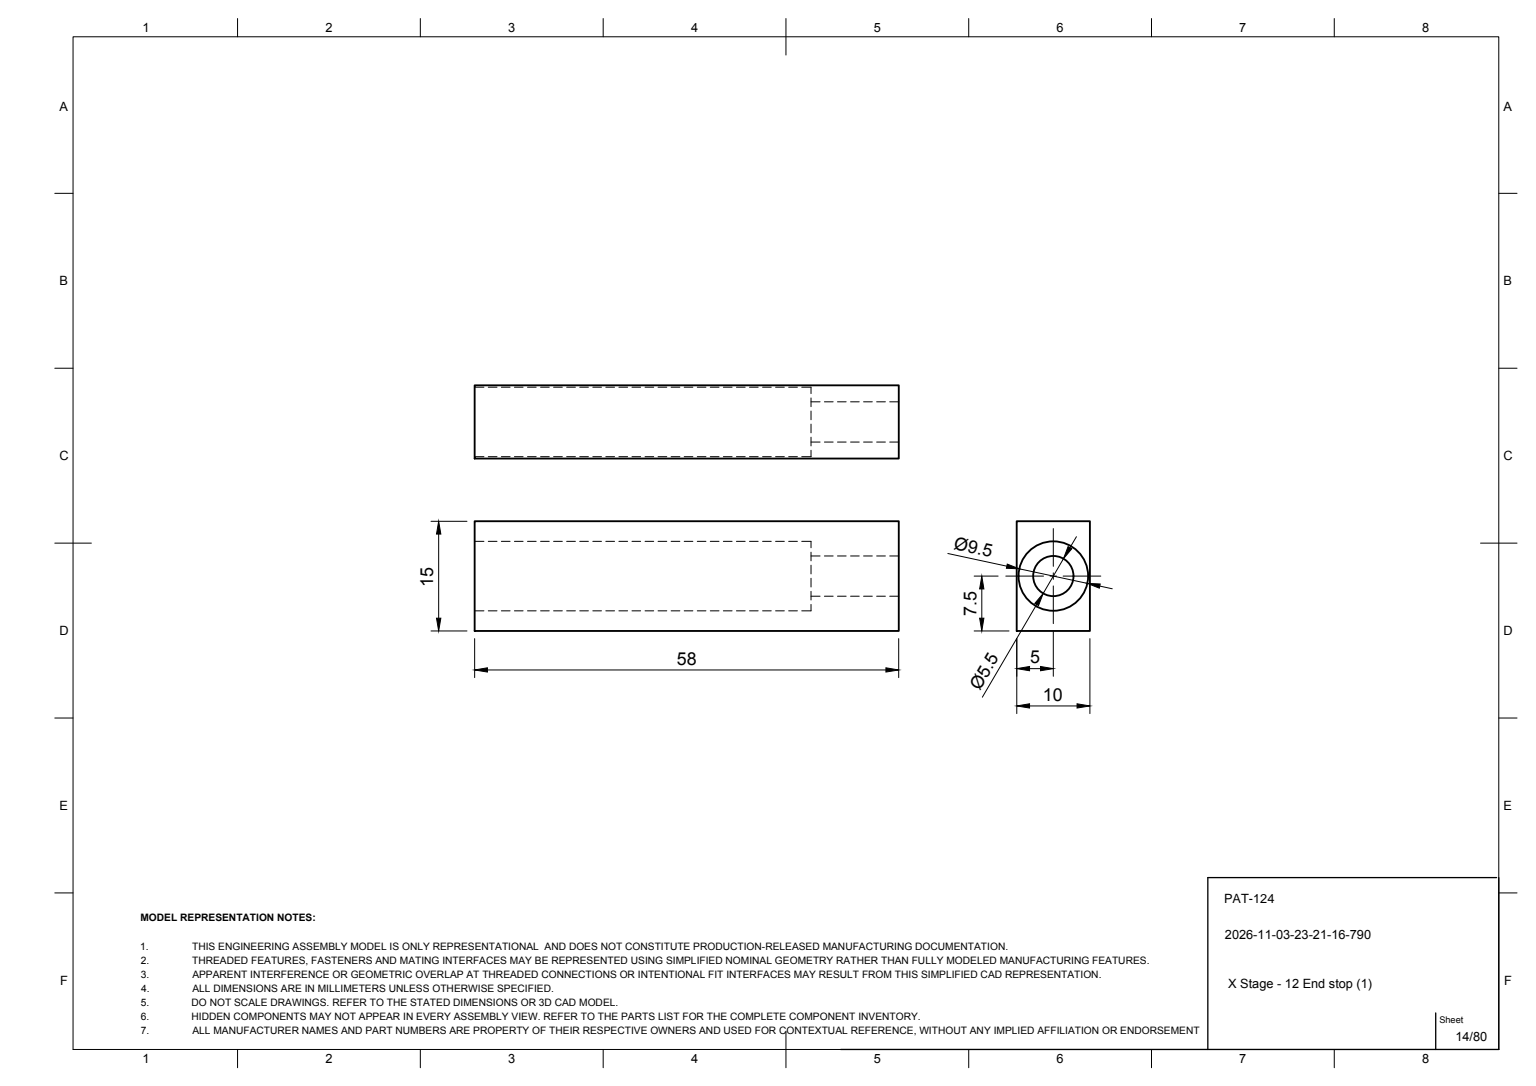
ISO-10303-21;
HEADER;
/* Generated by software containing ST-Developer
 * from STEP Tools, Inc. (www.steptools.com) 
 */

FILE_DESCRIPTION(
/* description */ ('XY cross-slide table'),
/* implementation_level */ '2;1');

FILE_NAME(
/* name */ 'X Stage - 12 End stop (1).step',
/* time_stamp */ '2026-10-28T03:22:46-07:00',
/* author */ (''),
/* organization */ (''),
/* preprocessor_version */ 'ST-DEVELOPER v20.2',
/* originating_system */ 'Autodesk Translation Framework v15.17.0.0',
/* authorisation */ '');

FILE_SCHEMA (('AUTOMOTIVE_DESIGN { 1 0 10303 214 3 1 1 }'));
ENDSEC;

DATA;
#10=MECHANICAL_DESIGN_GEOMETRIC_PRESENTATION_REPRESENTATION('',(#1679),#62984);
#1513=SHAPE_REPRESENTATION_RELATIONSHIP('SRR','None',#63361,#1596);
#1596=ADVANCED_BREP_SHAPE_REPRESENTATION('',(#1792),#62898);
#1679=STYLED_ITEM('',(#63905),#1792);
#1792=MANIFOLD_SOLID_BREP('Body1',#22973);
#1968=FACE_BOUND('',#4378,.T.);
#1969=FACE_BOUND('',#4385,.T.);
#1970=FACE_BOUND('',#4387,.T.);
#2356=PLANE('',#24232);
#2357=PLANE('',#24236);
#2358=PLANE('',#24237);
#2359=PLANE('',#24238);
#2360=PLANE('',#24239);
#2361=PLANE('',#24240);
#2362=PLANE('',#24241);
#2981=FACE_OUTER_BOUND('',#4376,.T.);
#2982=FACE_OUTER_BOUND('',#4377,.T.);
#2983=FACE_OUTER_BOUND('',#4379,.T.);
#2984=FACE_OUTER_BOUND('',#4380,.T.);
#2985=FACE_OUTER_BOUND('',#4381,.T.);
#2986=FACE_OUTER_BOUND('',#4382,.T.);
#2987=FACE_OUTER_BOUND('',#4383,.T.);
#2988=FACE_OUTER_BOUND('',#4384,.T.);
#2989=FACE_OUTER_BOUND('',#4386,.T.);
#4376=EDGE_LOOP('',(#15398,#15399,#15400,#15401));
#4377=EDGE_LOOP('',(#15402));
#4378=EDGE_LOOP('',(#15403));
#4379=EDGE_LOOP('',(#15404,#15405,#15406,#15407));
#4380=EDGE_LOOP('',(#15408,#15409,#15410,#15411));
#4381=EDGE_LOOP('',(#15412,#15413,#15414,#15415));
#4382=EDGE_LOOP('',(#15416,#15417,#15418,#15419));
#4383=EDGE_LOOP('',(#15420,#15421,#15422,#15423));
#4384=EDGE_LOOP('',(#15424,#15425,#15426,#15427));
#4385=EDGE_LOOP('',(#15428));
#4386=EDGE_LOOP('',(#15429,#15430,#15431,#15432));
#4387=EDGE_LOOP('',(#15433));
#6049=LINE('',#33408,#7536);
#6050=LINE('',#33416,#7537);
#6051=LINE('',#33420,#7538);
#6052=LINE('',#33422,#7539);
#6053=LINE('',#33424,#7540);
#6054=LINE('',#33425,#7541);
#6055=LINE('',#33428,#7542);
#6056=LINE('',#33430,#7543);
#6057=LINE('',#33431,#7544);
#6058=LINE('',#33434,#7545);
#6059=LINE('',#33436,#7546);
#6060=LINE('',#33437,#7547);
#6061=LINE('',#33439,#7548);
#6062=LINE('',#33440,#7549);
#7536=VECTOR('',#27066,0.475000000000001);
#7537=VECTOR('',#27077,0.274999999999999);
#7538=VECTOR('',#27080,1.);
#7539=VECTOR('',#27081,1.);
#7540=VECTOR('',#27082,1.);
#7541=VECTOR('',#27083,1.);
#7542=VECTOR('',#27086,1.);
#7543=VECTOR('',#27087,1.);
#7544=VECTOR('',#27088,1.);
#7545=VECTOR('',#27091,1.);
#7546=VECTOR('',#27092,1.);
#7547=VECTOR('',#27093,1.);
#7548=VECTOR('',#27096,1.);
#7549=VECTOR('',#27097,1.);
#8984=CIRCLE('',#24230,0.475000000000001);
#8985=CIRCLE('',#24231,0.475000000000001);
#8986=CIRCLE('',#24233,0.274999999999999);
#8987=CIRCLE('',#24235,0.274999999999999);
#9935=VERTEX_POINT('',#33405);
#9936=VERTEX_POINT('',#33407);
#9937=VERTEX_POINT('',#33411);
#9938=VERTEX_POINT('',#33414);
#9939=VERTEX_POINT('',#33418);
#9940=VERTEX_POINT('',#33419);
#9941=VERTEX_POINT('',#33421);
#9942=VERTEX_POINT('',#33423);
#9943=VERTEX_POINT('',#33427);
#9944=VERTEX_POINT('',#33429);
#9945=VERTEX_POINT('',#33433);
#9946=VERTEX_POINT('',#33435);
#12083=EDGE_CURVE('',#9935,#9935,#8984,.T.);
#12084=EDGE_CURVE('',#9935,#9936,#6049,.T.);
#12085=EDGE_CURVE('',#9936,#9936,#8985,.T.);
#12086=EDGE_CURVE('',#9937,#9937,#8986,.T.);
#12087=EDGE_CURVE('',#9938,#9938,#8987,.T.);
#12088=EDGE_CURVE('',#9938,#9937,#6050,.T.);
#12089=EDGE_CURVE('',#9939,#9940,#6051,.T.);
#12090=EDGE_CURVE('',#9940,#9941,#6052,.T.);
#12091=EDGE_CURVE('',#9942,#9941,#6053,.T.);
#12092=EDGE_CURVE('',#9939,#9942,#6054,.T.);
#12093=EDGE_CURVE('',#9943,#9939,#6055,.T.);
#12094=EDGE_CURVE('',#9944,#9942,#6056,.T.);
#12095=EDGE_CURVE('',#9943,#9944,#6057,.T.);
#12096=EDGE_CURVE('',#9945,#9943,#6058,.T.);
#12097=EDGE_CURVE('',#9946,#9944,#6059,.T.);
#12098=EDGE_CURVE('',#9945,#9946,#6060,.T.);
#12099=EDGE_CURVE('',#9940,#9945,#6061,.T.);
#12100=EDGE_CURVE('',#9941,#9946,#6062,.T.);
#15398=ORIENTED_EDGE('',*,*,#12083,.F.);
#15399=ORIENTED_EDGE('',*,*,#12084,.T.);
#15400=ORIENTED_EDGE('',*,*,#12085,.F.);
#15401=ORIENTED_EDGE('',*,*,#12084,.F.);
#15402=ORIENTED_EDGE('',*,*,#12083,.T.);
#15403=ORIENTED_EDGE('',*,*,#12086,.F.);
#15404=ORIENTED_EDGE('',*,*,#12087,.F.);
#15405=ORIENTED_EDGE('',*,*,#12088,.T.);
#15406=ORIENTED_EDGE('',*,*,#12086,.T.);
#15407=ORIENTED_EDGE('',*,*,#12088,.F.);
#15408=ORIENTED_EDGE('',*,*,#12089,.T.);
#15409=ORIENTED_EDGE('',*,*,#12090,.T.);
#15410=ORIENTED_EDGE('',*,*,#12091,.F.);
#15411=ORIENTED_EDGE('',*,*,#12092,.F.);
#15412=ORIENTED_EDGE('',*,*,#12093,.T.);
#15413=ORIENTED_EDGE('',*,*,#12092,.T.);
#15414=ORIENTED_EDGE('',*,*,#12094,.F.);
#15415=ORIENTED_EDGE('',*,*,#12095,.F.);
#15416=ORIENTED_EDGE('',*,*,#12096,.T.);
#15417=ORIENTED_EDGE('',*,*,#12095,.T.);
#15418=ORIENTED_EDGE('',*,*,#12097,.F.);
#15419=ORIENTED_EDGE('',*,*,#12098,.F.);
#15420=ORIENTED_EDGE('',*,*,#12099,.T.);
#15421=ORIENTED_EDGE('',*,*,#12098,.T.);
#15422=ORIENTED_EDGE('',*,*,#12100,.F.);
#15423=ORIENTED_EDGE('',*,*,#12090,.F.);
#15424=ORIENTED_EDGE('',*,*,#12100,.T.);
#15425=ORIENTED_EDGE('',*,*,#12097,.T.);
#15426=ORIENTED_EDGE('',*,*,#12094,.T.);
#15427=ORIENTED_EDGE('',*,*,#12091,.T.);
#15428=ORIENTED_EDGE('',*,*,#12085,.T.);
#15429=ORIENTED_EDGE('',*,*,#12099,.F.);
#15430=ORIENTED_EDGE('',*,*,#12089,.F.);
#15431=ORIENTED_EDGE('',*,*,#12093,.F.);
#15432=ORIENTED_EDGE('',*,*,#12096,.F.);
#15433=ORIENTED_EDGE('',*,*,#12087,.T.);
#21092=CYLINDRICAL_SURFACE('',#24229,0.475000000000001);
#21093=CYLINDRICAL_SURFACE('',#24234,0.274999999999999);
#21762=ADVANCED_FACE('',(#2981),#21092,.F.);
#21763=ADVANCED_FACE('',(#2982,#1968),#2356,.T.);
#21764=ADVANCED_FACE('',(#2983),#21093,.F.);
#21765=ADVANCED_FACE('',(#2984),#2357,.T.);
#21766=ADVANCED_FACE('',(#2985),#2358,.T.);
#21767=ADVANCED_FACE('',(#2986),#2359,.T.);
#21768=ADVANCED_FACE('',(#2987),#2360,.T.);
#21769=ADVANCED_FACE('',(#2988,#1969),#2361,.T.);
#21770=ADVANCED_FACE('',(#2989,#1970),#2362,.F.);
#22973=CLOSED_SHELL('',(#21762,#21763,#21764,#21765,#21766,#21767,#21768,
#21769,#21770));
#24228=AXIS2_PLACEMENT_3D('',#33403,#27060,#27061);
#24229=AXIS2_PLACEMENT_3D('',#33404,#27062,#27063);
#24230=AXIS2_PLACEMENT_3D('',#33406,#27064,#27065);
#24231=AXIS2_PLACEMENT_3D('',#33409,#27067,#27068);
#24232=AXIS2_PLACEMENT_3D('',#33410,#27069,#27070);
#24233=AXIS2_PLACEMENT_3D('',#33412,#27071,#27072);
#24234=AXIS2_PLACEMENT_3D('',#33413,#27073,#27074);
#24235=AXIS2_PLACEMENT_3D('',#33415,#27075,#27076);
#24236=AXIS2_PLACEMENT_3D('',#33417,#27078,#27079);
#24237=AXIS2_PLACEMENT_3D('',#33426,#27084,#27085);
#24238=AXIS2_PLACEMENT_3D('',#33432,#27089,#27090);
#24239=AXIS2_PLACEMENT_3D('',#33438,#27094,#27095);
#24240=AXIS2_PLACEMENT_3D('',#33441,#27098,#27099);
#24241=AXIS2_PLACEMENT_3D('',#33442,#27100,#27101);
#27060=DIRECTION('axis',(0.,0.,1.));
#27061=DIRECTION('refdir',(1.,0.,0.));
#27062=DIRECTION('center_axis',(0.,0.,1.));
#27063=DIRECTION('ref_axis',(1.,0.,0.));
#27064=DIRECTION('center_axis',(0.,0.,1.));
#27065=DIRECTION('ref_axis',(1.,0.,0.));
#27066=DIRECTION('',(0.,0.,1.));
#27067=DIRECTION('center_axis',(0.,0.,-1.));
#27068=DIRECTION('ref_axis',(1.,0.,0.));
#27069=DIRECTION('center_axis',(0.,0.,1.));
#27070=DIRECTION('ref_axis',(1.,0.,0.));
#27071=DIRECTION('center_axis',(0.,0.,1.));
#27072=DIRECTION('ref_axis',(1.,0.,0.));
#27073=DIRECTION('center_axis',(0.,0.,1.));
#27074=DIRECTION('ref_axis',(1.,0.,0.));
#27075=DIRECTION('center_axis',(0.,0.,1.));
#27076=DIRECTION('ref_axis',(1.,0.,0.));
#27077=DIRECTION('',(0.,0.,1.));
#27078=DIRECTION('center_axis',(0.,1.,0.));
#27079=DIRECTION('ref_axis',(-1.,0.,0.));
#27080=DIRECTION('',(-1.,0.,0.));
#27081=DIRECTION('',(0.,0.,1.));
#27082=DIRECTION('',(-1.,0.,0.));
#27083=DIRECTION('',(0.,0.,1.));
#27084=DIRECTION('center_axis',(1.,0.,0.));
#27085=DIRECTION('ref_axis',(0.,1.,0.));
#27086=DIRECTION('',(0.,1.,0.));
#27087=DIRECTION('',(0.,1.,0.));
#27088=DIRECTION('',(0.,0.,1.));
#27089=DIRECTION('center_axis',(0.,-1.,0.));
#27090=DIRECTION('ref_axis',(1.,0.,0.));
#27091=DIRECTION('',(1.,0.,0.));
#27092=DIRECTION('',(1.,0.,0.));
#27093=DIRECTION('',(0.,0.,1.));
#27094=DIRECTION('center_axis',(-1.,0.,0.));
#27095=DIRECTION('ref_axis',(0.,-1.,0.));
#27096=DIRECTION('',(0.,-1.,0.));
#27097=DIRECTION('',(0.,-1.,0.));
#27098=DIRECTION('center_axis',(0.,0.,1.));
#27099=DIRECTION('ref_axis',(1.,0.,0.));
#27100=DIRECTION('center_axis',(0.,0.,1.));
#27101=DIRECTION('ref_axis',(1.,0.,0.));
#33403=CARTESIAN_POINT('',(0.,0.,0.));
#33404=CARTESIAN_POINT('Origin',(23.5,-9.25,2.4));
#33405=CARTESIAN_POINT('',(23.025,-9.25,2.4));
#33406=CARTESIAN_POINT('Origin',(23.5,-9.25,2.4));
#33407=CARTESIAN_POINT('',(23.025,-9.25,7.));
#33408=CARTESIAN_POINT('',(23.025,-9.25,2.4));
#33409=CARTESIAN_POINT('Origin',(23.5,-9.25,7.));
#33410=CARTESIAN_POINT('Origin',(23.5,-9.25,2.4));
#33411=CARTESIAN_POINT('',(23.225,-9.25,2.4));
#33412=CARTESIAN_POINT('Origin',(23.5,-9.25,2.4));
#33413=CARTESIAN_POINT('Origin',(23.5,-9.25,1.1));
#33414=CARTESIAN_POINT('',(23.225,-9.25,1.2));
#33415=CARTESIAN_POINT('Origin',(23.5,-9.25,1.2));
#33416=CARTESIAN_POINT('',(23.225,-9.25,1.1));
#33417=CARTESIAN_POINT('Origin',(24.,-8.5,1.2));
#33418=CARTESIAN_POINT('',(24.,-8.5,1.2));
#33419=CARTESIAN_POINT('',(23.,-8.5,1.2));
#33420=CARTESIAN_POINT('',(24.,-8.5,1.2));
#33421=CARTESIAN_POINT('',(23.,-8.5,7.));
#33422=CARTESIAN_POINT('',(23.,-8.5,1.2));
#33423=CARTESIAN_POINT('',(24.,-8.5,7.));
#33424=CARTESIAN_POINT('',(24.,-8.5,7.));
#33425=CARTESIAN_POINT('',(24.,-8.5,1.2));
#33426=CARTESIAN_POINT('Origin',(24.,-10.,1.2));
#33427=CARTESIAN_POINT('',(24.,-10.,1.2));
#33428=CARTESIAN_POINT('',(24.,-10.,1.2));
#33429=CARTESIAN_POINT('',(24.,-10.,7.));
#33430=CARTESIAN_POINT('',(24.,-10.,7.));
#33431=CARTESIAN_POINT('',(24.,-10.,1.2));
#33432=CARTESIAN_POINT('Origin',(23.,-10.,1.2));
#33433=CARTESIAN_POINT('',(23.,-10.,1.2));
#33434=CARTESIAN_POINT('',(23.,-10.,1.2));
#33435=CARTESIAN_POINT('',(23.,-10.,7.));
#33436=CARTESIAN_POINT('',(23.,-10.,7.));
#33437=CARTESIAN_POINT('',(23.,-10.,1.2));
#33438=CARTESIAN_POINT('Origin',(23.,-8.5,1.2));
#33439=CARTESIAN_POINT('',(23.,-8.5,1.2));
#33440=CARTESIAN_POINT('',(23.,-8.5,7.));
#33441=CARTESIAN_POINT('Origin',(23.5,-9.25,7.));
#33442=CARTESIAN_POINT('Origin',(23.5,-9.25,1.2));
#62799=UNCERTAINTY_MEASURE_WITH_UNIT(LENGTH_MEASURE(0.001),#62985,
'DISTANCE_ACCURACY_VALUE',
'Maximum model space distance between geometric entities at asserted c
onnectivities');
#62885=UNCERTAINTY_MEASURE_WITH_UNIT(LENGTH_MEASURE(0.001),#62985,
'DISTANCE_ACCURACY_VALUE',
'Maximum model space distance between geometric entities at asserted c
onnectivities');
#62898=(
GEOMETRIC_REPRESENTATION_CONTEXT(3)
GLOBAL_UNCERTAINTY_ASSIGNED_CONTEXT((#62799))
GLOBAL_UNIT_ASSIGNED_CONTEXT((#62985,#62987,#62988))
REPRESENTATION_CONTEXT('','3D')
);
#62984=(
GEOMETRIC_REPRESENTATION_CONTEXT(3)
GLOBAL_UNCERTAINTY_ASSIGNED_CONTEXT((#62885))
GLOBAL_UNIT_ASSIGNED_CONTEXT((#62985,#62987,#62988))
REPRESENTATION_CONTEXT('','3D')
);
#62985=(
LENGTH_UNIT()
NAMED_UNIT(*)
SI_UNIT(.CENTI.,.METRE.)
);
#62987=(
NAMED_UNIT(*)
PLANE_ANGLE_UNIT()
SI_UNIT($,.RADIAN.)
);
#62988=(
NAMED_UNIT(*)
SI_UNIT($,.STERADIAN.)
SOLID_ANGLE_UNIT()
);
#63001=SHAPE_DEFINITION_REPRESENTATION(#63099,#63361);
#63099=PRODUCT_DEFINITION_SHAPE('',$,#63460);
#63361=SHAPE_REPRESENTATION('',(#24228),#62898);
#63447=PRODUCT_DEFINITION_CONTEXT('part definition',#63743,'design');
#63460=PRODUCT_DEFINITION('X Stage - 12 End stop (1)',
'X Stage - 12 End stop (1)',#63558,#63447);
#63558=PRODUCT_DEFINITION_FORMATION('',$,#63757);
#63743=APPLICATION_CONTEXT(
'Core Data for Automotive Mechanical Design Process');
#63744=PRODUCT_CONTEXT('part definition',#63743,'mechanical');
#63757=PRODUCT('X Stage - 12 End stop (1)','X Stage - 12 End stop (1)',
'X Stage - 12 End stop (1)',(#63744));
#63899=COLOUR_RGB('Sky Blue',0.24,0.69,0.87);
#63900=FILL_AREA_STYLE_COLOUR('',#63899);
#63901=FILL_AREA_STYLE('',(#63900));
#63902=SURFACE_STYLE_FILL_AREA(#63901);
#63903=SURFACE_SIDE_STYLE('',(#63902));
#63904=SURFACE_STYLE_USAGE(.BOTH.,#63903);
#63905=PRESENTATION_STYLE_ASSIGNMENT((#63904));
ENDSEC;
END-ISO-10303-21;
